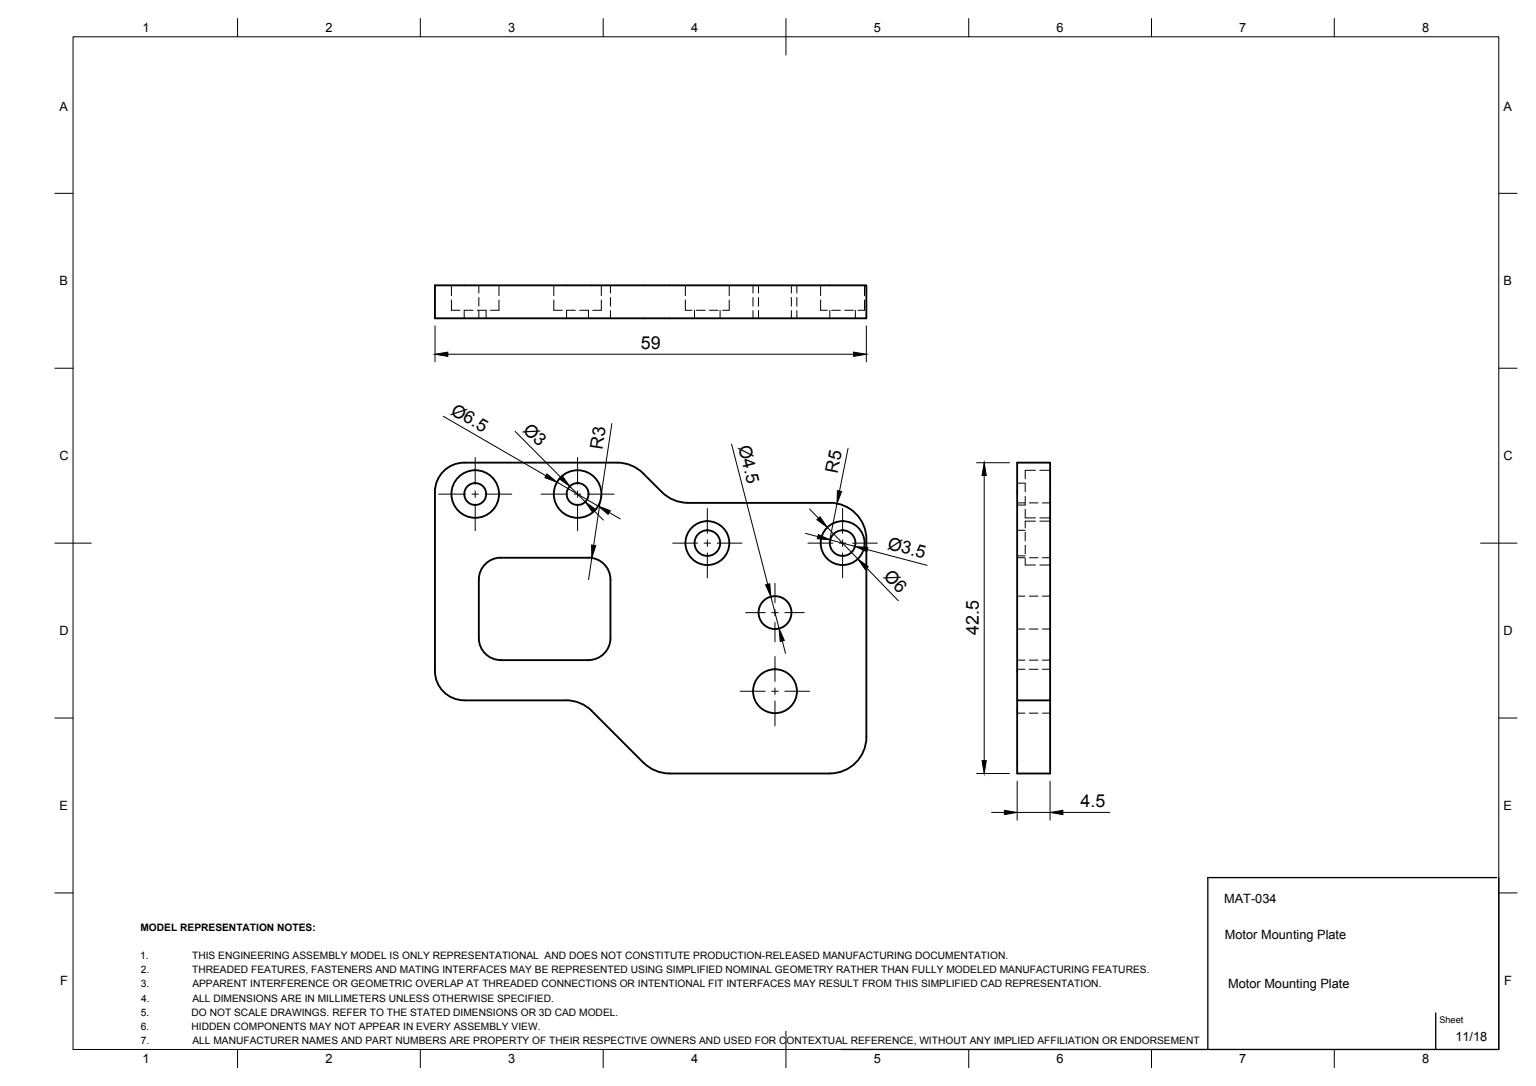
ISO-10303-21;
HEADER;
/* Generated by software containing ST-Developer
 * from STEP Tools, Inc. (www.steptools.com) 
 */

FILE_DESCRIPTION(
/* description */ ('STEP AP214'),
/* implementation_level */ '2;1');

FILE_NAME(
/* name */ 'Motor Mounting Plate.step',
/* time_stamp */ '2026-11-14T09:24:36-08:00',
/* author */ (''),
/* organization */ (''),
/* preprocessor_version */ 'ST-DEVELOPER v20.2',
/* originating_system */ 'Autodesk Translation Framework v15.17.0.0',
/* authorisation */ '');

FILE_SCHEMA (('AUTOMOTIVE_DESIGN { 1 0 10303 214 3 1 1 }'));
ENDSEC;

DATA;
#10=MECHANICAL_DESIGN_GEOMETRIC_PRESENTATION_REPRESENTATION('',(#207),#18867);
#175=SHAPE_REPRESENTATION_RELATIONSHIP('SRR','None',#18939,#191);
#191=ADVANCED_BREP_SHAPE_REPRESENTATION('',(#231),#18855);
#207=STYLED_ITEM('',(#19026),#231);
#231=MANIFOLD_SOLID_BREP('Body1',#10962);
#301=FACE_BOUND('',#1568,.T.);
#302=FACE_BOUND('',#1569,.T.);
#303=FACE_BOUND('',#1570,.T.);
#304=FACE_BOUND('',#1571,.T.);
#305=FACE_BOUND('',#1572,.T.);
#306=FACE_BOUND('',#1573,.T.);
#307=FACE_BOUND('',#1574,.T.);
#308=FACE_BOUND('',#1576,.T.);
#309=FACE_BOUND('',#1578,.T.);
#310=FACE_BOUND('',#1580,.T.);
#311=FACE_BOUND('',#1581,.T.);
#312=FACE_BOUND('',#1582,.T.);
#313=FACE_BOUND('',#1583,.T.);
#314=FACE_BOUND('',#1584,.T.);
#315=FACE_BOUND('',#1585,.T.);
#316=FACE_BOUND('',#1586,.T.);
#317=FACE_BOUND('',#1588,.T.);
#318=FACE_BOUND('',#1590,.T.);
#495=PLANE('',#11457);
#496=PLANE('',#11458);
#497=PLANE('',#11459);
#498=PLANE('',#11466);
#499=PLANE('',#11470);
#500=PLANE('',#11474);
#501=PLANE('',#11478);
#502=PLANE('',#11482);
#503=PLANE('',#11483);
#504=PLANE('',#11484);
#505=PLANE('',#11485);
#506=PLANE('',#11486);
#507=PLANE('',#11505);
#508=PLANE('',#11506);
#509=PLANE('',#11507);
#510=PLANE('',#11508);
#511=PLANE('',#11509);
#512=PLANE('',#11510);
#887=FACE_OUTER_BOUND('',#1533,.T.);
#888=FACE_OUTER_BOUND('',#1534,.T.);
#889=FACE_OUTER_BOUND('',#1535,.T.);
#890=FACE_OUTER_BOUND('',#1536,.T.);
#891=FACE_OUTER_BOUND('',#1537,.T.);
#892=FACE_OUTER_BOUND('',#1538,.T.);
#893=FACE_OUTER_BOUND('',#1539,.T.);
#894=FACE_OUTER_BOUND('',#1540,.T.);
#895=FACE_OUTER_BOUND('',#1541,.T.);
#896=FACE_OUTER_BOUND('',#1542,.T.);
#897=FACE_OUTER_BOUND('',#1543,.T.);
#898=FACE_OUTER_BOUND('',#1544,.T.);
#899=FACE_OUTER_BOUND('',#1545,.T.);
#900=FACE_OUTER_BOUND('',#1546,.T.);
#901=FACE_OUTER_BOUND('',#1547,.T.);
#902=FACE_OUTER_BOUND('',#1548,.T.);
#903=FACE_OUTER_BOUND('',#1549,.T.);
#904=FACE_OUTER_BOUND('',#1550,.T.);
#905=FACE_OUTER_BOUND('',#1551,.T.);
#906=FACE_OUTER_BOUND('',#1552,.T.);
#907=FACE_OUTER_BOUND('',#1553,.T.);
#908=FACE_OUTER_BOUND('',#1554,.T.);
#909=FACE_OUTER_BOUND('',#1555,.T.);
#910=FACE_OUTER_BOUND('',#1556,.T.);
#911=FACE_OUTER_BOUND('',#1557,.T.);
#912=FACE_OUTER_BOUND('',#1558,.T.);
#913=FACE_OUTER_BOUND('',#1559,.T.);
#914=FACE_OUTER_BOUND('',#1560,.T.);
#915=FACE_OUTER_BOUND('',#1561,.T.);
#916=FACE_OUTER_BOUND('',#1562,.T.);
#917=FACE_OUTER_BOUND('',#1563,.T.);
#918=FACE_OUTER_BOUND('',#1564,.T.);
#919=FACE_OUTER_BOUND('',#1565,.T.);
#920=FACE_OUTER_BOUND('',#1566,.T.);
#921=FACE_OUTER_BOUND('',#1567,.T.);
#922=FACE_OUTER_BOUND('',#1575,.T.);
#923=FACE_OUTER_BOUND('',#1577,.T.);
#924=FACE_OUTER_BOUND('',#1579,.T.);
#925=FACE_OUTER_BOUND('',#1587,.T.);
#926=FACE_OUTER_BOUND('',#1589,.T.);
#1533=EDGE_LOOP('',(#7916,#7917,#7918,#7919));
#1534=EDGE_LOOP('',(#7920,#7921,#7922,#7923));
#1535=EDGE_LOOP('',(#7924,#7925,#7926,#7927));
#1536=EDGE_LOOP('',(#7928,#7929,#7930,#7931));
#1537=EDGE_LOOP('',(#7932,#7933,#7934,#7935));
#1538=EDGE_LOOP('',(#7936,#7937,#7938,#7939));
#1539=EDGE_LOOP('',(#7940,#7941,#7942,#7943));
#1540=EDGE_LOOP('',(#7944,#7945,#7946,#7947));
#1541=EDGE_LOOP('',(#7948,#7949,#7950,#7951));
#1542=EDGE_LOOP('',(#7952,#7953,#7954,#7955));
#1543=EDGE_LOOP('',(#7956,#7957,#7958,#7959));
#1544=EDGE_LOOP('',(#7960,#7961,#7962,#7963));
#1545=EDGE_LOOP('',(#7964,#7965,#7966,#7967));
#1546=EDGE_LOOP('',(#7968,#7969,#7970,#7971));
#1547=EDGE_LOOP('',(#7972,#7973,#7974,#7975));
#1548=EDGE_LOOP('',(#7976,#7977,#7978,#7979));
#1549=EDGE_LOOP('',(#7980,#7981,#7982,#7983));
#1550=EDGE_LOOP('',(#7984,#7985,#7986,#7987));
#1551=EDGE_LOOP('',(#7988,#7989,#7990,#7991));
#1552=EDGE_LOOP('',(#7992,#7993,#7994,#7995));
#1553=EDGE_LOOP('',(#7996,#7997,#7998,#7999));
#1554=EDGE_LOOP('',(#8000,#8001,#8002,#8003));
#1555=EDGE_LOOP('',(#8004,#8005,#8006,#8007));
#1556=EDGE_LOOP('',(#8008,#8009,#8010,#8011));
#1557=EDGE_LOOP('',(#8012,#8013,#8014,#8015));
#1558=EDGE_LOOP('',(#8016,#8017,#8018,#8019));
#1559=EDGE_LOOP('',(#8020,#8021,#8022,#8023));
#1560=EDGE_LOOP('',(#8024,#8025,#8026,#8027));
#1561=EDGE_LOOP('',(#8028,#8029,#8030,#8031));
#1562=EDGE_LOOP('',(#8032,#8033,#8034,#8035));
#1563=EDGE_LOOP('',(#8036,#8037,#8038,#8039));
#1564=EDGE_LOOP('',(#8040,#8041,#8042,#8043));
#1565=EDGE_LOOP('',(#8044,#8045,#8046,#8047));
#1566=EDGE_LOOP('',(#8048,#8049,#8050,#8051));
#1567=EDGE_LOOP('',(#8052,#8053,#8054,#8055,#8056,#8057,#8058,#8059,#8060,
#8061,#8062,#8063,#8064,#8065,#8066,#8067));
#1568=EDGE_LOOP('',(#8068,#8069,#8070,#8071,#8072,#8073,#8074,#8075));
#1569=EDGE_LOOP('',(#8076));
#1570=EDGE_LOOP('',(#8077));
#1571=EDGE_LOOP('',(#8078));
#1572=EDGE_LOOP('',(#8079));
#1573=EDGE_LOOP('',(#8080));
#1574=EDGE_LOOP('',(#8081));
#1575=EDGE_LOOP('',(#8082));
#1576=EDGE_LOOP('',(#8083));
#1577=EDGE_LOOP('',(#8084));
#1578=EDGE_LOOP('',(#8085));
#1579=EDGE_LOOP('',(#8086,#8087,#8088,#8089,#8090,#8091,#8092,#8093,#8094,
#8095,#8096,#8097,#8098,#8099,#8100,#8101));
#1580=EDGE_LOOP('',(#8102));
#1581=EDGE_LOOP('',(#8103));
#1582=EDGE_LOOP('',(#8104));
#1583=EDGE_LOOP('',(#8105));
#1584=EDGE_LOOP('',(#8106));
#1585=EDGE_LOOP('',(#8107));
#1586=EDGE_LOOP('',(#8108,#8109,#8110,#8111,#8112,#8113,#8114,#8115));
#1587=EDGE_LOOP('',(#8116));
#1588=EDGE_LOOP('',(#8117));
#1589=EDGE_LOOP('',(#8118));
#1590=EDGE_LOOP('',(#8119));
#2351=LINE('',#16449,#3365);
#2352=LINE('',#16455,#3366);
#2353=LINE('',#16461,#3367);
#2354=LINE('',#16467,#3368);
#2355=LINE('',#16473,#3369);
#2356=LINE('',#16479,#3370);
#2357=LINE('',#16485,#3371);
#2358=LINE('',#16491,#3372);
#2359=LINE('',#16497,#3373);
#2360=LINE('',#16503,#3374);
#2361=LINE('',#16508,#3375);
#2362=LINE('',#16510,#3376);
#2363=LINE('',#16512,#3377);
#2364=LINE('',#16513,#3378);
#2365=LINE('',#16517,#3379);
#2366=LINE('',#16519,#3380);
#2367=LINE('',#16521,#3381);
#2368=LINE('',#16522,#3382);
#2369=LINE('',#16526,#3383);
#2370=LINE('',#16528,#3384);
#2371=LINE('',#16530,#3385);
#2372=LINE('',#16531,#3386);
#2373=LINE('',#16541,#3387);
#2374=LINE('',#16543,#3388);
#2375=LINE('',#16545,#3389);
#2376=LINE('',#16546,#3390);
#2377=LINE('',#16551,#3391);
#2378=LINE('',#16555,#3392);
#2379=LINE('',#16557,#3393);
#2380=LINE('',#16558,#3394);
#2381=LINE('',#16563,#3395);
#2382=LINE('',#16567,#3396);
#2383=LINE('',#16569,#3397);
#2384=LINE('',#16570,#3398);
#2385=LINE('',#16575,#3399);
#2386=LINE('',#16579,#3400);
#2387=LINE('',#16581,#3401);
#2388=LINE('',#16582,#3402);
#2389=LINE('',#16589,#3403);
#2390=LINE('',#16591,#3404);
#2391=LINE('',#16593,#3405);
#2392=LINE('',#16594,#3406);
#2393=LINE('',#16598,#3407);
#2394=LINE('',#16600,#3408);
#2395=LINE('',#16602,#3409);
#2396=LINE('',#16603,#3410);
#2397=LINE('',#16607,#3411);
#2398=LINE('',#16609,#3412);
#2399=LINE('',#16611,#3413);
#2400=LINE('',#16612,#3414);
#2401=LINE('',#16616,#3415);
#2402=LINE('',#16618,#3416);
#2403=LINE('',#16620,#3417);
#2404=LINE('',#16621,#3418);
#2405=LINE('',#16625,#3419);
#2406=LINE('',#16627,#3420);
#2407=LINE('',#16629,#3421);
#2408=LINE('',#16630,#3422);
#3365=VECTOR('',#13147,3.);
#3366=VECTOR('',#13154,3.);
#3367=VECTOR('',#13161,3.25);
#3368=VECTOR('',#13168,3.25);
#3369=VECTOR('',#13175,2.25);
#3370=VECTOR('',#13182,1.75);
#3371=VECTOR('',#13189,1.75);
#3372=VECTOR('',#13196,3.);
#3373=VECTOR('',#13203,1.5);
#3374=VECTOR('',#13210,1.5);
#3375=VECTOR('',#13215,1000.);
#3376=VECTOR('',#13216,1000.);
#3377=VECTOR('',#13217,1000.);
#3378=VECTOR('',#13218,1000.);
#3379=VECTOR('',#13221,1000.);
#3380=VECTOR('',#13222,1000.);
#3381=VECTOR('',#13223,1000.);
#3382=VECTOR('',#13224,1000.);
#3383=VECTOR('',#13227,1000.);
#3384=VECTOR('',#13228,1000.);
#3385=VECTOR('',#13229,1000.);
#3386=VECTOR('',#13230,1000.);
#3387=VECTOR('',#13245,1000.);
#3388=VECTOR('',#13246,1000.);
#3389=VECTOR('',#13247,1000.);
#3390=VECTOR('',#13248,1000.);
#3391=VECTOR('',#13253,1000.);
#3392=VECTOR('',#13258,1000.);
#3393=VECTOR('',#13259,1000.);
#3394=VECTOR('',#13260,1000.);
#3395=VECTOR('',#13265,1000.);
#3396=VECTOR('',#13270,1000.);
#3397=VECTOR('',#13271,1000.);
#3398=VECTOR('',#13272,1000.);
#3399=VECTOR('',#13277,1000.);
#3400=VECTOR('',#13282,1000.);
#3401=VECTOR('',#13283,1000.);
#3402=VECTOR('',#13284,1000.);
#3403=VECTOR('',#13293,1000.);
#3404=VECTOR('',#13294,1000.);
#3405=VECTOR('',#13295,1000.);
#3406=VECTOR('',#13296,1000.);
#3407=VECTOR('',#13299,1000.);
#3408=VECTOR('',#13300,1000.);
#3409=VECTOR('',#13301,1000.);
#3410=VECTOR('',#13302,1000.);
#3411=VECTOR('',#13305,1000.);
#3412=VECTOR('',#13306,1000.);
#3413=VECTOR('',#13307,1000.);
#3414=VECTOR('',#13308,1000.);
#3415=VECTOR('',#13311,1000.);
#3416=VECTOR('',#13312,1000.);
#3417=VECTOR('',#13313,1000.);
#3418=VECTOR('',#13314,1000.);
#3419=VECTOR('',#13317,1000.);
#3420=VECTOR('',#13318,1000.);
#3421=VECTOR('',#13319,1000.);
#3422=VECTOR('',#13320,1000.);
#4171=CIRCLE('',#11428,3.);
#4172=CIRCLE('',#11429,3.);
#4173=CIRCLE('',#11431,3.);
#4174=CIRCLE('',#11432,3.);
#4175=CIRCLE('',#11434,3.25);
#4176=CIRCLE('',#11435,3.25);
#4177=CIRCLE('',#11437,3.25);
#4178=CIRCLE('',#11438,3.25);
#4179=CIRCLE('',#11440,2.25);
#4180=CIRCLE('',#11441,2.25);
#4181=CIRCLE('',#11443,1.75);
#4182=CIRCLE('',#11444,1.75);
#4183=CIRCLE('',#11446,1.75);
#4184=CIRCLE('',#11447,1.75);
#4185=CIRCLE('',#11449,3.);
#4186=CIRCLE('',#11450,3.);
#4187=CIRCLE('',#11452,1.5);
#4188=CIRCLE('',#11453,1.5);
#4189=CIRCLE('',#11455,1.5);
#4190=CIRCLE('',#11456,1.5);
#4191=CIRCLE('',#11461,4.);
#4192=CIRCLE('',#11462,4.);
#4193=CIRCLE('',#11464,4.);
#4194=CIRCLE('',#11465,4.);
#4195=CIRCLE('',#11468,3.);
#4196=CIRCLE('',#11469,3.);
#4197=CIRCLE('',#11472,3.);
#4198=CIRCLE('',#11473,3.);
#4199=CIRCLE('',#11476,3.);
#4200=CIRCLE('',#11477,3.);
#4201=CIRCLE('',#11480,3.);
#4202=CIRCLE('',#11481,3.);
#4203=CIRCLE('',#11488,5.);
#4204=CIRCLE('',#11489,5.);
#4205=CIRCLE('',#11491,5.);
#4206=CIRCLE('',#11492,5.);
#4207=CIRCLE('',#11494,5.);
#4208=CIRCLE('',#11495,5.);
#4209=CIRCLE('',#11497,5.);
#4210=CIRCLE('',#11498,5.);
#4211=CIRCLE('',#11500,5.);
#4212=CIRCLE('',#11501,5.);
#4213=CIRCLE('',#11503,5.);
#4214=CIRCLE('',#11504,5.);
#4842=VERTEX_POINT('',#16446);
#4843=VERTEX_POINT('',#16448);
#4844=VERTEX_POINT('',#16452);
#4845=VERTEX_POINT('',#16454);
#4846=VERTEX_POINT('',#16458);
#4847=VERTEX_POINT('',#16460);
#4848=VERTEX_POINT('',#16464);
#4849=VERTEX_POINT('',#16466);
#4850=VERTEX_POINT('',#16470);
#4851=VERTEX_POINT('',#16472);
#4852=VERTEX_POINT('',#16476);
#4853=VERTEX_POINT('',#16478);
#4854=VERTEX_POINT('',#16482);
#4855=VERTEX_POINT('',#16484);
#4856=VERTEX_POINT('',#16488);
#4857=VERTEX_POINT('',#16490);
#4858=VERTEX_POINT('',#16494);
#4859=VERTEX_POINT('',#16496);
#4860=VERTEX_POINT('',#16500);
#4861=VERTEX_POINT('',#16502);
#4862=VERTEX_POINT('',#16506);
#4863=VERTEX_POINT('',#16507);
#4864=VERTEX_POINT('',#16509);
#4865=VERTEX_POINT('',#16511);
#4866=VERTEX_POINT('',#16515);
#4867=VERTEX_POINT('',#16516);
#4868=VERTEX_POINT('',#16518);
#4869=VERTEX_POINT('',#16520);
#4870=VERTEX_POINT('',#16524);
#4871=VERTEX_POINT('',#16525);
#4872=VERTEX_POINT('',#16527);
#4873=VERTEX_POINT('',#16529);
#4874=VERTEX_POINT('',#16539);
#4875=VERTEX_POINT('',#16540);
#4876=VERTEX_POINT('',#16542);
#4877=VERTEX_POINT('',#16544);
#4878=VERTEX_POINT('',#16548);
#4879=VERTEX_POINT('',#16550);
#4880=VERTEX_POINT('',#16554);
#4881=VERTEX_POINT('',#16556);
#4882=VERTEX_POINT('',#16560);
#4883=VERTEX_POINT('',#16562);
#4884=VERTEX_POINT('',#16566);
#4885=VERTEX_POINT('',#16568);
#4886=VERTEX_POINT('',#16572);
#4887=VERTEX_POINT('',#16574);
#4888=VERTEX_POINT('',#16578);
#4889=VERTEX_POINT('',#16580);
#4890=VERTEX_POINT('',#16587);
#4891=VERTEX_POINT('',#16588);
#4892=VERTEX_POINT('',#16590);
#4893=VERTEX_POINT('',#16592);
#4894=VERTEX_POINT('',#16596);
#4895=VERTEX_POINT('',#16597);
#4896=VERTEX_POINT('',#16599);
#4897=VERTEX_POINT('',#16601);
#4898=VERTEX_POINT('',#16605);
#4899=VERTEX_POINT('',#16606);
#4900=VERTEX_POINT('',#16608);
#4901=VERTEX_POINT('',#16610);
#4902=VERTEX_POINT('',#16614);
#4903=VERTEX_POINT('',#16615);
#4904=VERTEX_POINT('',#16617);
#4905=VERTEX_POINT('',#16619);
#4906=VERTEX_POINT('',#16623);
#4907=VERTEX_POINT('',#16624);
#4908=VERTEX_POINT('',#16626);
#4909=VERTEX_POINT('',#16628);
#5991=EDGE_CURVE('',#4842,#4842,#4171,.T.);
#5992=EDGE_CURVE('',#4842,#4843,#2351,.T.);
#5993=EDGE_CURVE('',#4843,#4843,#4172,.T.);
#5994=EDGE_CURVE('',#4844,#4844,#4173,.T.);
#5995=EDGE_CURVE('',#4844,#4845,#2352,.T.);
#5996=EDGE_CURVE('',#4845,#4845,#4174,.T.);
#5997=EDGE_CURVE('',#4846,#4846,#4175,.T.);
#5998=EDGE_CURVE('',#4846,#4847,#2353,.T.);
#5999=EDGE_CURVE('',#4847,#4847,#4176,.T.);
#6000=EDGE_CURVE('',#4848,#4848,#4177,.T.);
#6001=EDGE_CURVE('',#4848,#4849,#2354,.T.);
#6002=EDGE_CURVE('',#4849,#4849,#4178,.T.);
#6003=EDGE_CURVE('',#4850,#4850,#4179,.T.);
#6004=EDGE_CURVE('',#4850,#4851,#2355,.T.);
#6005=EDGE_CURVE('',#4851,#4851,#4180,.T.);
#6006=EDGE_CURVE('',#4852,#4852,#4181,.T.);
#6007=EDGE_CURVE('',#4852,#4853,#2356,.T.);
#6008=EDGE_CURVE('',#4853,#4853,#4182,.T.);
#6009=EDGE_CURVE('',#4854,#4854,#4183,.T.);
#6010=EDGE_CURVE('',#4854,#4855,#2357,.T.);
#6011=EDGE_CURVE('',#4855,#4855,#4184,.T.);
#6012=EDGE_CURVE('',#4856,#4856,#4185,.T.);
#6013=EDGE_CURVE('',#4856,#4857,#2358,.T.);
#6014=EDGE_CURVE('',#4857,#4857,#4186,.T.);
#6015=EDGE_CURVE('',#4858,#4858,#4187,.T.);
#6016=EDGE_CURVE('',#4858,#4859,#2359,.T.);
#6017=EDGE_CURVE('',#4859,#4859,#4188,.T.);
#6018=EDGE_CURVE('',#4860,#4860,#4189,.T.);
#6019=EDGE_CURVE('',#4860,#4861,#2360,.T.);
#6020=EDGE_CURVE('',#4861,#4861,#4190,.T.);
#6021=EDGE_CURVE('',#4862,#4863,#2361,.T.);
#6022=EDGE_CURVE('',#4862,#4864,#2362,.T.);
#6023=EDGE_CURVE('',#4865,#4864,#2363,.T.);
#6024=EDGE_CURVE('',#4865,#4863,#2364,.T.);
#6025=EDGE_CURVE('',#4866,#4867,#2365,.T.);
#6026=EDGE_CURVE('',#4866,#4868,#2366,.T.);
#6027=EDGE_CURVE('',#4869,#4868,#2367,.T.);
#6028=EDGE_CURVE('',#4869,#4867,#2368,.T.);
#6029=EDGE_CURVE('',#4870,#4871,#2369,.T.);
#6030=EDGE_CURVE('',#4870,#4872,#2370,.T.);
#6031=EDGE_CURVE('',#4873,#4872,#2371,.T.);
#6032=EDGE_CURVE('',#4873,#4871,#2372,.T.);
#6033=EDGE_CURVE('',#4871,#4866,#4191,.T.);
#6034=EDGE_CURVE('',#4868,#4873,#4192,.T.);
#6035=EDGE_CURVE('',#4867,#4862,#4193,.T.);
#6036=EDGE_CURVE('',#4864,#4869,#4194,.T.);
#6037=EDGE_CURVE('',#4874,#4875,#2373,.T.);
#6038=EDGE_CURVE('',#4874,#4876,#2374,.T.);
#6039=EDGE_CURVE('',#4876,#4877,#2375,.T.);
#6040=EDGE_CURVE('',#4875,#4877,#2376,.T.);
#6041=EDGE_CURVE('',#4878,#4876,#4195,.T.);
#6042=EDGE_CURVE('',#4878,#4879,#2377,.T.);
#6043=EDGE_CURVE('',#4879,#4877,#4196,.T.);
#6044=EDGE_CURVE('',#4878,#4880,#2378,.T.);
#6045=EDGE_CURVE('',#4880,#4881,#2379,.T.);
#6046=EDGE_CURVE('',#4879,#4881,#2380,.T.);
#6047=EDGE_CURVE('',#4882,#4880,#4197,.T.);
#6048=EDGE_CURVE('',#4882,#4883,#2381,.T.);
#6049=EDGE_CURVE('',#4883,#4881,#4198,.T.);
#6050=EDGE_CURVE('',#4884,#4882,#2382,.T.);
#6051=EDGE_CURVE('',#4884,#4885,#2383,.T.);
#6052=EDGE_CURVE('',#4885,#4883,#2384,.T.);
#6053=EDGE_CURVE('',#4886,#4884,#4199,.T.);
#6054=EDGE_CURVE('',#4886,#4887,#2385,.T.);
#6055=EDGE_CURVE('',#4887,#4885,#4200,.T.);
#6056=EDGE_CURVE('',#4888,#4886,#2386,.T.);
#6057=EDGE_CURVE('',#4888,#4889,#2387,.T.);
#6058=EDGE_CURVE('',#4889,#4887,#2388,.T.);
#6059=EDGE_CURVE('',#4874,#4888,#4201,.T.);
#6060=EDGE_CURVE('',#4875,#4889,#4202,.T.);
#6061=EDGE_CURVE('',#4890,#4891,#2389,.T.);
#6062=EDGE_CURVE('',#4892,#4891,#2390,.T.);
#6063=EDGE_CURVE('',#4892,#4893,#2391,.T.);
#6064=EDGE_CURVE('',#4890,#4893,#2392,.T.);
#6065=EDGE_CURVE('',#4894,#4895,#2393,.T.);
#6066=EDGE_CURVE('',#4896,#4895,#2394,.T.);
#6067=EDGE_CURVE('',#4896,#4897,#2395,.T.);
#6068=EDGE_CURVE('',#4894,#4897,#2396,.T.);
#6069=EDGE_CURVE('',#4898,#4899,#2397,.T.);
#6070=EDGE_CURVE('',#4900,#4899,#2398,.T.);
#6071=EDGE_CURVE('',#4900,#4901,#2399,.T.);
#6072=EDGE_CURVE('',#4898,#4901,#2400,.T.);
#6073=EDGE_CURVE('',#4902,#4903,#2401,.T.);
#6074=EDGE_CURVE('',#4904,#4903,#2402,.T.);
#6075=EDGE_CURVE('',#4904,#4905,#2403,.T.);
#6076=EDGE_CURVE('',#4902,#4905,#2404,.T.);
#6077=EDGE_CURVE('',#4906,#4907,#2405,.T.);
#6078=EDGE_CURVE('',#4908,#4907,#2406,.T.);
#6079=EDGE_CURVE('',#4908,#4909,#2407,.T.);
#6080=EDGE_CURVE('',#4906,#4909,#2408,.T.);
#6081=EDGE_CURVE('',#4863,#4908,#4203,.T.);
#6082=EDGE_CURVE('',#4909,#4865,#4204,.T.);
#6083=EDGE_CURVE('',#4907,#4904,#4205,.T.);
#6084=EDGE_CURVE('',#4905,#4906,#4206,.T.);
#6085=EDGE_CURVE('',#4903,#4900,#4207,.T.);
#6086=EDGE_CURVE('',#4901,#4902,#4208,.T.);
#6087=EDGE_CURVE('',#4899,#4892,#4209,.T.);
#6088=EDGE_CURVE('',#4893,#4898,#4210,.T.);
#6089=EDGE_CURVE('',#4891,#4896,#4211,.T.);
#6090=EDGE_CURVE('',#4897,#4890,#4212,.T.);
#6091=EDGE_CURVE('',#4895,#4870,#4213,.T.);
#6092=EDGE_CURVE('',#4872,#4894,#4214,.T.);
#7916=ORIENTED_EDGE('',*,*,#5991,.F.);
#7917=ORIENTED_EDGE('',*,*,#5992,.T.);
#7918=ORIENTED_EDGE('',*,*,#5993,.T.);
#7919=ORIENTED_EDGE('',*,*,#5992,.F.);
#7920=ORIENTED_EDGE('',*,*,#5994,.F.);
#7921=ORIENTED_EDGE('',*,*,#5995,.T.);
#7922=ORIENTED_EDGE('',*,*,#5996,.T.);
#7923=ORIENTED_EDGE('',*,*,#5995,.F.);
#7924=ORIENTED_EDGE('',*,*,#5997,.F.);
#7925=ORIENTED_EDGE('',*,*,#5998,.T.);
#7926=ORIENTED_EDGE('',*,*,#5999,.T.);
#7927=ORIENTED_EDGE('',*,*,#5998,.F.);
#7928=ORIENTED_EDGE('',*,*,#6000,.F.);
#7929=ORIENTED_EDGE('',*,*,#6001,.T.);
#7930=ORIENTED_EDGE('',*,*,#6002,.T.);
#7931=ORIENTED_EDGE('',*,*,#6001,.F.);
#7932=ORIENTED_EDGE('',*,*,#6003,.F.);
#7933=ORIENTED_EDGE('',*,*,#6004,.T.);
#7934=ORIENTED_EDGE('',*,*,#6005,.F.);
#7935=ORIENTED_EDGE('',*,*,#6004,.F.);
#7936=ORIENTED_EDGE('',*,*,#6006,.F.);
#7937=ORIENTED_EDGE('',*,*,#6007,.T.);
#7938=ORIENTED_EDGE('',*,*,#6008,.T.);
#7939=ORIENTED_EDGE('',*,*,#6007,.F.);
#7940=ORIENTED_EDGE('',*,*,#6009,.F.);
#7941=ORIENTED_EDGE('',*,*,#6010,.T.);
#7942=ORIENTED_EDGE('',*,*,#6011,.T.);
#7943=ORIENTED_EDGE('',*,*,#6010,.F.);
#7944=ORIENTED_EDGE('',*,*,#6012,.F.);
#7945=ORIENTED_EDGE('',*,*,#6013,.T.);
#7946=ORIENTED_EDGE('',*,*,#6014,.T.);
#7947=ORIENTED_EDGE('',*,*,#6013,.F.);
#7948=ORIENTED_EDGE('',*,*,#6015,.F.);
#7949=ORIENTED_EDGE('',*,*,#6016,.T.);
#7950=ORIENTED_EDGE('',*,*,#6017,.T.);
#7951=ORIENTED_EDGE('',*,*,#6016,.F.);
#7952=ORIENTED_EDGE('',*,*,#6018,.F.);
#7953=ORIENTED_EDGE('',*,*,#6019,.T.);
#7954=ORIENTED_EDGE('',*,*,#6020,.T.);
#7955=ORIENTED_EDGE('',*,*,#6019,.F.);
#7956=ORIENTED_EDGE('',*,*,#6021,.F.);
#7957=ORIENTED_EDGE('',*,*,#6022,.T.);
#7958=ORIENTED_EDGE('',*,*,#6023,.F.);
#7959=ORIENTED_EDGE('',*,*,#6024,.T.);
#7960=ORIENTED_EDGE('',*,*,#6025,.F.);
#7961=ORIENTED_EDGE('',*,*,#6026,.T.);
#7962=ORIENTED_EDGE('',*,*,#6027,.F.);
#7963=ORIENTED_EDGE('',*,*,#6028,.T.);
#7964=ORIENTED_EDGE('',*,*,#6029,.F.);
#7965=ORIENTED_EDGE('',*,*,#6030,.T.);
#7966=ORIENTED_EDGE('',*,*,#6031,.F.);
#7967=ORIENTED_EDGE('',*,*,#6032,.T.);
#7968=ORIENTED_EDGE('',*,*,#6026,.F.);
#7969=ORIENTED_EDGE('',*,*,#6033,.F.);
#7970=ORIENTED_EDGE('',*,*,#6032,.F.);
#7971=ORIENTED_EDGE('',*,*,#6034,.F.);
#7972=ORIENTED_EDGE('',*,*,#6022,.F.);
#7973=ORIENTED_EDGE('',*,*,#6035,.F.);
#7974=ORIENTED_EDGE('',*,*,#6028,.F.);
#7975=ORIENTED_EDGE('',*,*,#6036,.F.);
#7976=ORIENTED_EDGE('',*,*,#6037,.F.);
#7977=ORIENTED_EDGE('',*,*,#6038,.T.);
#7978=ORIENTED_EDGE('',*,*,#6039,.T.);
#7979=ORIENTED_EDGE('',*,*,#6040,.F.);
#7980=ORIENTED_EDGE('',*,*,#6041,.F.);
#7981=ORIENTED_EDGE('',*,*,#6042,.T.);
#7982=ORIENTED_EDGE('',*,*,#6043,.T.);
#7983=ORIENTED_EDGE('',*,*,#6039,.F.);
#7984=ORIENTED_EDGE('',*,*,#6042,.F.);
#7985=ORIENTED_EDGE('',*,*,#6044,.T.);
#7986=ORIENTED_EDGE('',*,*,#6045,.T.);
#7987=ORIENTED_EDGE('',*,*,#6046,.F.);
#7988=ORIENTED_EDGE('',*,*,#6047,.F.);
#7989=ORIENTED_EDGE('',*,*,#6048,.T.);
#7990=ORIENTED_EDGE('',*,*,#6049,.T.);
#7991=ORIENTED_EDGE('',*,*,#6045,.F.);
#7992=ORIENTED_EDGE('',*,*,#6050,.F.);
#7993=ORIENTED_EDGE('',*,*,#6051,.T.);
#7994=ORIENTED_EDGE('',*,*,#6052,.T.);
#7995=ORIENTED_EDGE('',*,*,#6048,.F.);
#7996=ORIENTED_EDGE('',*,*,#6053,.F.);
#7997=ORIENTED_EDGE('',*,*,#6054,.T.);
#7998=ORIENTED_EDGE('',*,*,#6055,.T.);
#7999=ORIENTED_EDGE('',*,*,#6051,.F.);
#8000=ORIENTED_EDGE('',*,*,#6056,.F.);
#8001=ORIENTED_EDGE('',*,*,#6057,.T.);
#8002=ORIENTED_EDGE('',*,*,#6058,.T.);
#8003=ORIENTED_EDGE('',*,*,#6054,.F.);
#8004=ORIENTED_EDGE('',*,*,#6059,.F.);
#8005=ORIENTED_EDGE('',*,*,#6037,.T.);
#8006=ORIENTED_EDGE('',*,*,#6060,.T.);
#8007=ORIENTED_EDGE('',*,*,#6057,.F.);
#8008=ORIENTED_EDGE('',*,*,#6061,.T.);
#8009=ORIENTED_EDGE('',*,*,#6062,.F.);
#8010=ORIENTED_EDGE('',*,*,#6063,.T.);
#8011=ORIENTED_EDGE('',*,*,#6064,.F.);
#8012=ORIENTED_EDGE('',*,*,#6065,.T.);
#8013=ORIENTED_EDGE('',*,*,#6066,.F.);
#8014=ORIENTED_EDGE('',*,*,#6067,.T.);
#8015=ORIENTED_EDGE('',*,*,#6068,.F.);
#8016=ORIENTED_EDGE('',*,*,#6069,.T.);
#8017=ORIENTED_EDGE('',*,*,#6070,.F.);
#8018=ORIENTED_EDGE('',*,*,#6071,.T.);
#8019=ORIENTED_EDGE('',*,*,#6072,.F.);
#8020=ORIENTED_EDGE('',*,*,#6073,.T.);
#8021=ORIENTED_EDGE('',*,*,#6074,.F.);
#8022=ORIENTED_EDGE('',*,*,#6075,.T.);
#8023=ORIENTED_EDGE('',*,*,#6076,.F.);
#8024=ORIENTED_EDGE('',*,*,#6077,.T.);
#8025=ORIENTED_EDGE('',*,*,#6078,.F.);
#8026=ORIENTED_EDGE('',*,*,#6079,.T.);
#8027=ORIENTED_EDGE('',*,*,#6080,.F.);
#8028=ORIENTED_EDGE('',*,*,#6079,.F.);
#8029=ORIENTED_EDGE('',*,*,#6081,.F.);
#8030=ORIENTED_EDGE('',*,*,#6024,.F.);
#8031=ORIENTED_EDGE('',*,*,#6082,.F.);
#8032=ORIENTED_EDGE('',*,*,#6083,.F.);
#8033=ORIENTED_EDGE('',*,*,#6077,.F.);
#8034=ORIENTED_EDGE('',*,*,#6084,.F.);
#8035=ORIENTED_EDGE('',*,*,#6075,.F.);
#8036=ORIENTED_EDGE('',*,*,#6071,.F.);
#8037=ORIENTED_EDGE('',*,*,#6085,.F.);
#8038=ORIENTED_EDGE('',*,*,#6073,.F.);
#8039=ORIENTED_EDGE('',*,*,#6086,.F.);
#8040=ORIENTED_EDGE('',*,*,#6063,.F.);
#8041=ORIENTED_EDGE('',*,*,#6087,.F.);
#8042=ORIENTED_EDGE('',*,*,#6069,.F.);
#8043=ORIENTED_EDGE('',*,*,#6088,.F.);
#8044=ORIENTED_EDGE('',*,*,#6067,.F.);
#8045=ORIENTED_EDGE('',*,*,#6089,.F.);
#8046=ORIENTED_EDGE('',*,*,#6061,.F.);
#8047=ORIENTED_EDGE('',*,*,#6090,.F.);
#8048=ORIENTED_EDGE('',*,*,#6091,.F.);
#8049=ORIENTED_EDGE('',*,*,#6065,.F.);
#8050=ORIENTED_EDGE('',*,*,#6092,.F.);
#8051=ORIENTED_EDGE('',*,*,#6030,.F.);
#8052=ORIENTED_EDGE('',*,*,#6080,.T.);
#8053=ORIENTED_EDGE('',*,*,#6082,.T.);
#8054=ORIENTED_EDGE('',*,*,#6023,.T.);
#8055=ORIENTED_EDGE('',*,*,#6036,.T.);
#8056=ORIENTED_EDGE('',*,*,#6027,.T.);
#8057=ORIENTED_EDGE('',*,*,#6034,.T.);
#8058=ORIENTED_EDGE('',*,*,#6031,.T.);
#8059=ORIENTED_EDGE('',*,*,#6092,.T.);
#8060=ORIENTED_EDGE('',*,*,#6068,.T.);
#8061=ORIENTED_EDGE('',*,*,#6090,.T.);
#8062=ORIENTED_EDGE('',*,*,#6064,.T.);
#8063=ORIENTED_EDGE('',*,*,#6088,.T.);
#8064=ORIENTED_EDGE('',*,*,#6072,.T.);
#8065=ORIENTED_EDGE('',*,*,#6086,.T.);
#8066=ORIENTED_EDGE('',*,*,#6076,.T.);
#8067=ORIENTED_EDGE('',*,*,#6084,.T.);
#8068=ORIENTED_EDGE('',*,*,#6060,.F.);
#8069=ORIENTED_EDGE('',*,*,#6040,.T.);
#8070=ORIENTED_EDGE('',*,*,#6043,.F.);
#8071=ORIENTED_EDGE('',*,*,#6046,.T.);
#8072=ORIENTED_EDGE('',*,*,#6049,.F.);
#8073=ORIENTED_EDGE('',*,*,#6052,.F.);
#8074=ORIENTED_EDGE('',*,*,#6055,.F.);
#8075=ORIENTED_EDGE('',*,*,#6058,.F.);
#8076=ORIENTED_EDGE('',*,*,#5993,.F.);
#8077=ORIENTED_EDGE('',*,*,#5996,.F.);
#8078=ORIENTED_EDGE('',*,*,#6003,.T.);
#8079=ORIENTED_EDGE('',*,*,#6014,.F.);
#8080=ORIENTED_EDGE('',*,*,#5999,.F.);
#8081=ORIENTED_EDGE('',*,*,#6002,.F.);
#8082=ORIENTED_EDGE('',*,*,#6000,.T.);
#8083=ORIENTED_EDGE('',*,*,#6020,.F.);
#8084=ORIENTED_EDGE('',*,*,#5997,.T.);
#8085=ORIENTED_EDGE('',*,*,#6017,.F.);
#8086=ORIENTED_EDGE('',*,*,#6035,.T.);
#8087=ORIENTED_EDGE('',*,*,#6021,.T.);
#8088=ORIENTED_EDGE('',*,*,#6081,.T.);
#8089=ORIENTED_EDGE('',*,*,#6078,.T.);
#8090=ORIENTED_EDGE('',*,*,#6083,.T.);
#8091=ORIENTED_EDGE('',*,*,#6074,.T.);
#8092=ORIENTED_EDGE('',*,*,#6085,.T.);
#8093=ORIENTED_EDGE('',*,*,#6070,.T.);
#8094=ORIENTED_EDGE('',*,*,#6087,.T.);
#8095=ORIENTED_EDGE('',*,*,#6062,.T.);
#8096=ORIENTED_EDGE('',*,*,#6089,.T.);
#8097=ORIENTED_EDGE('',*,*,#6066,.T.);
#8098=ORIENTED_EDGE('',*,*,#6091,.T.);
#8099=ORIENTED_EDGE('',*,*,#6029,.T.);
#8100=ORIENTED_EDGE('',*,*,#6033,.T.);
#8101=ORIENTED_EDGE('',*,*,#6025,.T.);
#8102=ORIENTED_EDGE('',*,*,#6005,.T.);
#8103=ORIENTED_EDGE('',*,*,#6006,.T.);
#8104=ORIENTED_EDGE('',*,*,#6009,.T.);
#8105=ORIENTED_EDGE('',*,*,#6012,.T.);
#8106=ORIENTED_EDGE('',*,*,#6015,.T.);
#8107=ORIENTED_EDGE('',*,*,#6018,.T.);
#8108=ORIENTED_EDGE('',*,*,#6059,.T.);
#8109=ORIENTED_EDGE('',*,*,#6056,.T.);
#8110=ORIENTED_EDGE('',*,*,#6053,.T.);
#8111=ORIENTED_EDGE('',*,*,#6050,.T.);
#8112=ORIENTED_EDGE('',*,*,#6047,.T.);
#8113=ORIENTED_EDGE('',*,*,#6044,.F.);
#8114=ORIENTED_EDGE('',*,*,#6041,.T.);
#8115=ORIENTED_EDGE('',*,*,#6038,.F.);
#8116=ORIENTED_EDGE('',*,*,#5994,.T.);
#8117=ORIENTED_EDGE('',*,*,#6008,.F.);
#8118=ORIENTED_EDGE('',*,*,#5991,.T.);
#8119=ORIENTED_EDGE('',*,*,#6011,.F.);
#10198=CYLINDRICAL_SURFACE('',#11427,3.);
#10199=CYLINDRICAL_SURFACE('',#11430,3.);
#10200=CYLINDRICAL_SURFACE('',#11433,3.25);
#10201=CYLINDRICAL_SURFACE('',#11436,3.25);
#10202=CYLINDRICAL_SURFACE('',#11439,2.25);
#10203=CYLINDRICAL_SURFACE('',#11442,1.75);
#10204=CYLINDRICAL_SURFACE('',#11445,1.75);
#10205=CYLINDRICAL_SURFACE('',#11448,3.);
#10206=CYLINDRICAL_SURFACE('',#11451,1.5);
#10207=CYLINDRICAL_SURFACE('',#11454,1.5);
#10208=CYLINDRICAL_SURFACE('',#11460,4.);
#10209=CYLINDRICAL_SURFACE('',#11463,4.);
#10210=CYLINDRICAL_SURFACE('',#11467,3.);
#10211=CYLINDRICAL_SURFACE('',#11471,3.);
#10212=CYLINDRICAL_SURFACE('',#11475,3.);
#10213=CYLINDRICAL_SURFACE('',#11479,3.);
#10214=CYLINDRICAL_SURFACE('',#11487,5.);
#10215=CYLINDRICAL_SURFACE('',#11490,5.);
#10216=CYLINDRICAL_SURFACE('',#11493,5.);
#10217=CYLINDRICAL_SURFACE('',#11496,5.);
#10218=CYLINDRICAL_SURFACE('',#11499,5.);
#10219=CYLINDRICAL_SURFACE('',#11502,5.);
#10524=ADVANCED_FACE('',(#887),#10198,.F.);
#10525=ADVANCED_FACE('',(#888),#10199,.F.);
#10526=ADVANCED_FACE('',(#889),#10200,.F.);
#10527=ADVANCED_FACE('',(#890),#10201,.F.);
#10528=ADVANCED_FACE('',(#891),#10202,.F.);
#10529=ADVANCED_FACE('',(#892),#10203,.F.);
#10530=ADVANCED_FACE('',(#893),#10204,.F.);
#10531=ADVANCED_FACE('',(#894),#10205,.F.);
#10532=ADVANCED_FACE('',(#895),#10206,.F.);
#10533=ADVANCED_FACE('',(#896),#10207,.F.);
#10534=ADVANCED_FACE('',(#897),#495,.F.);
#10535=ADVANCED_FACE('',(#898),#496,.F.);
#10536=ADVANCED_FACE('',(#899),#497,.F.);
#10537=ADVANCED_FACE('',(#900),#10208,.T.);
#10538=ADVANCED_FACE('',(#901),#10209,.T.);
#10539=ADVANCED_FACE('',(#902),#498,.T.);
#10540=ADVANCED_FACE('',(#903),#10210,.F.);
#10541=ADVANCED_FACE('',(#904),#499,.T.);
#10542=ADVANCED_FACE('',(#905),#10211,.F.);
#10543=ADVANCED_FACE('',(#906),#500,.F.);
#10544=ADVANCED_FACE('',(#907),#10212,.F.);
#10545=ADVANCED_FACE('',(#908),#501,.F.);
#10546=ADVANCED_FACE('',(#909),#10213,.F.);
#10547=ADVANCED_FACE('',(#910),#502,.T.);
#10548=ADVANCED_FACE('',(#911),#503,.T.);
#10549=ADVANCED_FACE('',(#912),#504,.T.);
#10550=ADVANCED_FACE('',(#913),#505,.T.);
#10551=ADVANCED_FACE('',(#914),#506,.T.);
#10552=ADVANCED_FACE('',(#915),#10214,.T.);
#10553=ADVANCED_FACE('',(#916),#10215,.F.);
#10554=ADVANCED_FACE('',(#917),#10216,.T.);
#10555=ADVANCED_FACE('',(#918),#10217,.T.);
#10556=ADVANCED_FACE('',(#919),#10218,.T.);
#10557=ADVANCED_FACE('',(#920),#10219,.F.);
#10558=ADVANCED_FACE('',(#921,#301,#302,#303,#304,#305,#306,#307),#507,
 .T.);
#10559=ADVANCED_FACE('',(#922,#308),#508,.F.);
#10560=ADVANCED_FACE('',(#923,#309),#509,.F.);
#10561=ADVANCED_FACE('',(#924,#310,#311,#312,#313,#314,#315,#316),#510,
 .T.);
#10562=ADVANCED_FACE('',(#925,#317),#511,.F.);
#10563=ADVANCED_FACE('',(#926,#318),#512,.F.);
#10962=CLOSED_SHELL('',(#10524,#10525,#10526,#10527,#10528,#10529,#10530,
#10531,#10532,#10533,#10534,#10535,#10536,#10537,#10538,#10539,#10540,#10541,
#10542,#10543,#10544,#10545,#10546,#10547,#10548,#10549,#10550,#10551,#10552,
#10553,#10554,#10555,#10556,#10557,#10558,#10559,#10560,#10561,#10562,#10563));
#11426=AXIS2_PLACEMENT_3D('',#16444,#13141,#13142);
#11427=AXIS2_PLACEMENT_3D('',#16445,#13143,#13144);
#11428=AXIS2_PLACEMENT_3D('',#16447,#13145,#13146);
#11429=AXIS2_PLACEMENT_3D('',#16450,#13148,#13149);
#11430=AXIS2_PLACEMENT_3D('',#16451,#13150,#13151);
#11431=AXIS2_PLACEMENT_3D('',#16453,#13152,#13153);
#11432=AXIS2_PLACEMENT_3D('',#16456,#13155,#13156);
#11433=AXIS2_PLACEMENT_3D('',#16457,#13157,#13158);
#11434=AXIS2_PLACEMENT_3D('',#16459,#13159,#13160);
#11435=AXIS2_PLACEMENT_3D('',#16462,#13162,#13163);
#11436=AXIS2_PLACEMENT_3D('',#16463,#13164,#13165);
#11437=AXIS2_PLACEMENT_3D('',#16465,#13166,#13167);
#11438=AXIS2_PLACEMENT_3D('',#16468,#13169,#13170);
#11439=AXIS2_PLACEMENT_3D('',#16469,#13171,#13172);
#11440=AXIS2_PLACEMENT_3D('',#16471,#13173,#13174);
#11441=AXIS2_PLACEMENT_3D('',#16474,#13176,#13177);
#11442=AXIS2_PLACEMENT_3D('',#16475,#13178,#13179);
#11443=AXIS2_PLACEMENT_3D('',#16477,#13180,#13181);
#11444=AXIS2_PLACEMENT_3D('',#16480,#13183,#13184);
#11445=AXIS2_PLACEMENT_3D('',#16481,#13185,#13186);
#11446=AXIS2_PLACEMENT_3D('',#16483,#13187,#13188);
#11447=AXIS2_PLACEMENT_3D('',#16486,#13190,#13191);
#11448=AXIS2_PLACEMENT_3D('',#16487,#13192,#13193);
#11449=AXIS2_PLACEMENT_3D('',#16489,#13194,#13195);
#11450=AXIS2_PLACEMENT_3D('',#16492,#13197,#13198);
#11451=AXIS2_PLACEMENT_3D('',#16493,#13199,#13200);
#11452=AXIS2_PLACEMENT_3D('',#16495,#13201,#13202);
#11453=AXIS2_PLACEMENT_3D('',#16498,#13204,#13205);
#11454=AXIS2_PLACEMENT_3D('',#16499,#13206,#13207);
#11455=AXIS2_PLACEMENT_3D('',#16501,#13208,#13209);
#11456=AXIS2_PLACEMENT_3D('',#16504,#13211,#13212);
#11457=AXIS2_PLACEMENT_3D('',#16505,#13213,#13214);
#11458=AXIS2_PLACEMENT_3D('',#16514,#13219,#13220);
#11459=AXIS2_PLACEMENT_3D('',#16523,#13225,#13226);
#11460=AXIS2_PLACEMENT_3D('',#16532,#13231,#13232);
#11461=AXIS2_PLACEMENT_3D('',#16533,#13233,#13234);
#11462=AXIS2_PLACEMENT_3D('',#16534,#13235,#13236);
#11463=AXIS2_PLACEMENT_3D('',#16535,#13237,#13238);
#11464=AXIS2_PLACEMENT_3D('',#16536,#13239,#13240);
#11465=AXIS2_PLACEMENT_3D('',#16537,#13241,#13242);
#11466=AXIS2_PLACEMENT_3D('',#16538,#13243,#13244);
#11467=AXIS2_PLACEMENT_3D('',#16547,#13249,#13250);
#11468=AXIS2_PLACEMENT_3D('',#16549,#13251,#13252);
#11469=AXIS2_PLACEMENT_3D('',#16552,#13254,#13255);
#11470=AXIS2_PLACEMENT_3D('',#16553,#13256,#13257);
#11471=AXIS2_PLACEMENT_3D('',#16559,#13261,#13262);
#11472=AXIS2_PLACEMENT_3D('',#16561,#13263,#13264);
#11473=AXIS2_PLACEMENT_3D('',#16564,#13266,#13267);
#11474=AXIS2_PLACEMENT_3D('',#16565,#13268,#13269);
#11475=AXIS2_PLACEMENT_3D('',#16571,#13273,#13274);
#11476=AXIS2_PLACEMENT_3D('',#16573,#13275,#13276);
#11477=AXIS2_PLACEMENT_3D('',#16576,#13278,#13279);
#11478=AXIS2_PLACEMENT_3D('',#16577,#13280,#13281);
#11479=AXIS2_PLACEMENT_3D('',#16583,#13285,#13286);
#11480=AXIS2_PLACEMENT_3D('',#16584,#13287,#13288);
#11481=AXIS2_PLACEMENT_3D('',#16585,#13289,#13290);
#11482=AXIS2_PLACEMENT_3D('',#16586,#13291,#13292);
#11483=AXIS2_PLACEMENT_3D('',#16595,#13297,#13298);
#11484=AXIS2_PLACEMENT_3D('',#16604,#13303,#13304);
#11485=AXIS2_PLACEMENT_3D('',#16613,#13309,#13310);
#11486=AXIS2_PLACEMENT_3D('',#16622,#13315,#13316);
#11487=AXIS2_PLACEMENT_3D('',#16631,#13321,#13322);
#11488=AXIS2_PLACEMENT_3D('',#16632,#13323,#13324);
#11489=AXIS2_PLACEMENT_3D('',#16633,#13325,#13326);
#11490=AXIS2_PLACEMENT_3D('',#16634,#13327,#13328);
#11491=AXIS2_PLACEMENT_3D('',#16635,#13329,#13330);
#11492=AXIS2_PLACEMENT_3D('',#16636,#13331,#13332);
#11493=AXIS2_PLACEMENT_3D('',#16637,#13333,#13334);
#11494=AXIS2_PLACEMENT_3D('',#16638,#13335,#13336);
#11495=AXIS2_PLACEMENT_3D('',#16639,#13337,#13338);
#11496=AXIS2_PLACEMENT_3D('',#16640,#13339,#13340);
#11497=AXIS2_PLACEMENT_3D('',#16641,#13341,#13342);
#11498=AXIS2_PLACEMENT_3D('',#16642,#13343,#13344);
#11499=AXIS2_PLACEMENT_3D('',#16643,#13345,#13346);
#11500=AXIS2_PLACEMENT_3D('',#16644,#13347,#13348);
#11501=AXIS2_PLACEMENT_3D('',#16645,#13349,#13350);
#11502=AXIS2_PLACEMENT_3D('',#16646,#13351,#13352);
#11503=AXIS2_PLACEMENT_3D('',#16647,#13353,#13354);
#11504=AXIS2_PLACEMENT_3D('',#16648,#13355,#13356);
#11505=AXIS2_PLACEMENT_3D('',#16649,#13357,#13358);
#11506=AXIS2_PLACEMENT_3D('',#16650,#13359,#13360);
#11507=AXIS2_PLACEMENT_3D('',#16651,#13361,#13362);
#11508=AXIS2_PLACEMENT_3D('',#16652,#13363,#13364);
#11509=AXIS2_PLACEMENT_3D('',#16653,#13365,#13366);
#11510=AXIS2_PLACEMENT_3D('',#16654,#13367,#13368);
#13141=DIRECTION('axis',(0.,0.,1.));
#13142=DIRECTION('refdir',(1.,0.,0.));
#13143=DIRECTION('center_axis',(0.,0.,1.));
#13144=DIRECTION('ref_axis',(1.,0.,0.));
#13145=DIRECTION('center_axis',(0.,0.,1.));
#13146=DIRECTION('ref_axis',(1.,0.,0.));
#13147=DIRECTION('',(0.,0.,1.));
#13148=DIRECTION('center_axis',(0.,0.,1.));
#13149=DIRECTION('ref_axis',(1.,0.,0.));
#13150=DIRECTION('center_axis',(0.,0.,1.));
#13151=DIRECTION('ref_axis',(1.,0.,0.));
#13152=DIRECTION('center_axis',(0.,0.,1.));
#13153=DIRECTION('ref_axis',(1.,0.,0.));
#13154=DIRECTION('',(0.,0.,1.));
#13155=DIRECTION('center_axis',(0.,0.,1.));
#13156=DIRECTION('ref_axis',(1.,0.,0.));
#13157=DIRECTION('center_axis',(0.,0.,1.));
#13158=DIRECTION('ref_axis',(1.,0.,0.));
#13159=DIRECTION('center_axis',(0.,0.,1.));
#13160=DIRECTION('ref_axis',(1.,0.,0.));
#13161=DIRECTION('',(0.,0.,1.));
#13162=DIRECTION('center_axis',(0.,0.,1.));
#13163=DIRECTION('ref_axis',(1.,0.,0.));
#13164=DIRECTION('center_axis',(0.,0.,1.));
#13165=DIRECTION('ref_axis',(1.,0.,0.));
#13166=DIRECTION('center_axis',(0.,0.,1.));
#13167=DIRECTION('ref_axis',(1.,0.,0.));
#13168=DIRECTION('',(0.,0.,1.));
#13169=DIRECTION('center_axis',(0.,0.,1.));
#13170=DIRECTION('ref_axis',(1.,0.,0.));
#13171=DIRECTION('center_axis',(0.,0.,-1.));
#13172=DIRECTION('ref_axis',(-1.,0.,0.));
#13173=DIRECTION('center_axis',(0.,0.,-1.));
#13174=DIRECTION('ref_axis',(-1.,0.,0.));
#13175=DIRECTION('',(0.,0.,-1.));
#13176=DIRECTION('center_axis',(0.,0.,1.));
#13177=DIRECTION('ref_axis',(-1.,0.,0.));
#13178=DIRECTION('center_axis',(0.,0.,1.));
#13179=DIRECTION('ref_axis',(1.,0.,0.));
#13180=DIRECTION('center_axis',(0.,0.,1.));
#13181=DIRECTION('ref_axis',(-1.,0.,0.));
#13182=DIRECTION('',(0.,0.,1.));
#13183=DIRECTION('center_axis',(0.,0.,1.));
#13184=DIRECTION('ref_axis',(-1.,0.,0.));
#13185=DIRECTION('center_axis',(0.,0.,1.));
#13186=DIRECTION('ref_axis',(1.,0.,0.));
#13187=DIRECTION('center_axis',(0.,0.,1.));
#13188=DIRECTION('ref_axis',(-1.,0.,0.));
#13189=DIRECTION('',(0.,0.,1.));
#13190=DIRECTION('center_axis',(0.,0.,1.));
#13191=DIRECTION('ref_axis',(-1.,0.,0.));
#13192=DIRECTION('center_axis',(0.,0.,1.));
#13193=DIRECTION('ref_axis',(1.,0.,0.));
#13194=DIRECTION('center_axis',(0.,0.,1.));
#13195=DIRECTION('ref_axis',(-1.,0.,0.));
#13196=DIRECTION('',(0.,0.,1.));
#13197=DIRECTION('center_axis',(0.,0.,1.));
#13198=DIRECTION('ref_axis',(1.,0.,0.));
#13199=DIRECTION('center_axis',(0.,0.,1.));
#13200=DIRECTION('ref_axis',(1.,0.,0.));
#13201=DIRECTION('center_axis',(0.,0.,1.));
#13202=DIRECTION('ref_axis',(-1.,0.,0.));
#13203=DIRECTION('',(0.,0.,1.));
#13204=DIRECTION('center_axis',(0.,0.,1.));
#13205=DIRECTION('ref_axis',(1.,0.,0.));
#13206=DIRECTION('center_axis',(0.,0.,1.));
#13207=DIRECTION('ref_axis',(1.,0.,0.));
#13208=DIRECTION('center_axis',(0.,0.,1.));
#13209=DIRECTION('ref_axis',(-1.,0.,0.));
#13210=DIRECTION('',(0.,0.,1.));
#13211=DIRECTION('center_axis',(0.,0.,1.));
#13212=DIRECTION('ref_axis',(1.,0.,0.));
#13213=DIRECTION('center_axis',(-1.,2.77555756156289E-16,0.));
#13214=DIRECTION('ref_axis',(-2.77555756156289E-16,-1.,0.));
#13215=DIRECTION('',(-3.31545529486744E-16,-1.,0.));
#13216=DIRECTION('',(0.,0.,1.));
#13217=DIRECTION('',(-4.78544407166016E-16,1.,0.));
#13218=DIRECTION('',(0.,0.,-1.));
#13219=DIRECTION('center_axis',(0.,-1.,0.));
#13220=DIRECTION('ref_axis',(0.,0.,-1.));
#13221=DIRECTION('',(1.,0.,0.));
#13222=DIRECTION('',(0.,0.,1.));
#13223=DIRECTION('',(-1.,0.,0.));
#13224=DIRECTION('',(0.,0.,-1.));
#13225=DIRECTION('center_axis',(1.,0.,0.));
#13226=DIRECTION('ref_axis',(0.,0.,-1.));
#13227=DIRECTION('',(0.,1.,0.));
#13228=DIRECTION('',(0.,0.,1.));
#13229=DIRECTION('',(0.,-1.,0.));
#13230=DIRECTION('',(0.,0.,-1.));
#13231=DIRECTION('center_axis',(0.,0.,-1.));
#13232=DIRECTION('ref_axis',(-1.,0.,0.));
#13233=DIRECTION('center_axis',(0.,0.,-1.));
#13234=DIRECTION('ref_axis',(-1.,0.,0.));
#13235=DIRECTION('center_axis',(0.,0.,1.));
#13236=DIRECTION('ref_axis',(1.,0.,0.));
#13237=DIRECTION('center_axis',(0.,0.,-1.));
#13238=DIRECTION('ref_axis',(-1.,0.,0.));
#13239=DIRECTION('center_axis',(0.,0.,-1.));
#13240=DIRECTION('ref_axis',(-1.,0.,0.));
#13241=DIRECTION('center_axis',(0.,0.,1.));
#13242=DIRECTION('ref_axis',(1.,0.,0.));
#13243=DIRECTION('center_axis',(0.,-1.,0.));
#13244=DIRECTION('ref_axis',(0.,0.,-1.));
#13245=DIRECTION('',(0.,0.,1.));
#13246=DIRECTION('',(1.,0.,0.));
#13247=DIRECTION('',(0.,0.,1.));
#13248=DIRECTION('',(1.,0.,0.));
#13249=DIRECTION('center_axis',(0.,0.,1.));
#13250=DIRECTION('ref_axis',(1.,0.,0.));
#13251=DIRECTION('center_axis',(0.,0.,1.));
#13252=DIRECTION('ref_axis',(-1.,0.,0.));
#13253=DIRECTION('',(0.,0.,1.));
#13254=DIRECTION('center_axis',(0.,0.,1.));
#13255=DIRECTION('ref_axis',(1.,0.,0.));
#13256=DIRECTION('center_axis',(-1.,-1.44560289664734E-16,0.));
#13257=DIRECTION('ref_axis',(1.44560289664734E-16,-1.,0.));
#13258=DIRECTION('',(1.44560289664734E-16,-1.,0.));
#13259=DIRECTION('',(0.,0.,1.));
#13260=DIRECTION('',(1.44560289664734E-16,-1.,0.));
#13261=DIRECTION('center_axis',(0.,0.,1.));
#13262=DIRECTION('ref_axis',(1.,0.,0.));
#13263=DIRECTION('center_axis',(0.,0.,1.));
#13264=DIRECTION('ref_axis',(-1.,1.15648231731787E-15,0.));
#13265=DIRECTION('',(0.,0.,1.));
#13266=DIRECTION('center_axis',(0.,0.,1.));
#13267=DIRECTION('ref_axis',(1.,0.,0.));
#13268=DIRECTION('center_axis',(0.,-1.,0.));
#13269=DIRECTION('ref_axis',(0.,0.,-1.));
#13270=DIRECTION('',(1.,0.,0.));
#13271=DIRECTION('',(0.,0.,1.));
#13272=DIRECTION('',(1.,0.,0.));
#13273=DIRECTION('center_axis',(0.,0.,1.));
#13274=DIRECTION('ref_axis',(1.,0.,0.));
#13275=DIRECTION('center_axis',(0.,0.,1.));
#13276=DIRECTION('ref_axis',(-1.,0.,0.));
#13277=DIRECTION('',(0.,0.,1.));
#13278=DIRECTION('center_axis',(0.,0.,1.));
#13279=DIRECTION('ref_axis',(1.,0.,0.));
#13280=DIRECTION('center_axis',(-1.,-1.44560289664734E-16,0.));
#13281=DIRECTION('ref_axis',(1.44560289664734E-16,-1.,0.));
#13282=DIRECTION('',(1.44560289664734E-16,-1.,0.));
#13283=DIRECTION('',(0.,0.,1.));
#13284=DIRECTION('',(1.44560289664734E-16,-1.,0.));
#13285=DIRECTION('center_axis',(0.,0.,1.));
#13286=DIRECTION('ref_axis',(1.,0.,0.));
#13287=DIRECTION('center_axis',(0.,0.,1.));
#13288=DIRECTION('ref_axis',(-1.,0.,0.));
#13289=DIRECTION('center_axis',(0.,0.,1.));
#13290=DIRECTION('ref_axis',(1.,0.,0.));
#13291=DIRECTION('center_axis',(-1.,-1.19636101791504E-16,0.));
#13292=DIRECTION('ref_axis',(1.19636101791504E-16,-1.,0.));
#13293=DIRECTION('',(0.,0.,-1.));
#13294=DIRECTION('',(0.,1.,0.));
#13295=DIRECTION('',(0.,0.,1.));
#13296=DIRECTION('',(1.19636101791504E-16,-1.,0.));
#13297=DIRECTION('center_axis',(-0.707106781186546,0.707106781186549,0.));
#13298=DIRECTION('ref_axis',(-0.707106781186549,-0.707106781186546,0.));
#13299=DIRECTION('',(0.,0.,-1.));
#13300=DIRECTION('',(0.707106781186549,0.707106781186546,0.));
#13301=DIRECTION('',(0.,0.,1.));
#13302=DIRECTION('',(-0.707106781186549,-0.707106781186546,0.));
#13303=DIRECTION('center_axis',(0.,-1.,0.));
#13304=DIRECTION('ref_axis',(0.,0.,-1.));
#13305=DIRECTION('',(0.,0.,-1.));
#13306=DIRECTION('',(-1.,6.42490176287706E-17,0.));
#13307=DIRECTION('',(0.,0.,1.));
#13308=DIRECTION('',(1.,0.,0.));
#13309=DIRECTION('center_axis',(1.,0.,0.));
#13310=DIRECTION('ref_axis',(0.,0.,-1.));
#13311=DIRECTION('',(0.,0.,-1.));
#13312=DIRECTION('',(0.,-1.,0.));
#13313=DIRECTION('',(0.,0.,1.));
#13314=DIRECTION('',(0.,1.,0.));
#13315=DIRECTION('center_axis',(0.707106781186547,-0.707106781186548,0.));
#13316=DIRECTION('ref_axis',(0.707106781186548,0.707106781186547,0.));
#13317=DIRECTION('',(0.,0.,-1.));
#13318=DIRECTION('',(-0.707106781186549,-0.707106781186546,0.));
#13319=DIRECTION('',(0.,0.,1.));
#13320=DIRECTION('',(0.707106781186548,0.707106781186547,0.));
#13321=DIRECTION('center_axis',(0.,0.,1.));
#13322=DIRECTION('ref_axis',(1.,0.,0.));
#13323=DIRECTION('center_axis',(0.,0.,-1.));
#13324=DIRECTION('ref_axis',(-1.,0.,0.));
#13325=DIRECTION('center_axis',(0.,0.,1.));
#13326=DIRECTION('ref_axis',(1.,0.,0.));
#13327=DIRECTION('center_axis',(0.,0.,-1.));
#13328=DIRECTION('ref_axis',(-1.,0.,0.));
#13329=DIRECTION('center_axis',(0.,0.,1.));
#13330=DIRECTION('ref_axis',(-1.,0.,0.));
#13331=DIRECTION('center_axis',(0.,0.,-1.));
#13332=DIRECTION('ref_axis',(1.,1.73472347597681E-15,0.));
#13333=DIRECTION('center_axis',(0.,0.,1.));
#13334=DIRECTION('ref_axis',(1.,0.,0.));
#13335=DIRECTION('center_axis',(0.,0.,-1.));
#13336=DIRECTION('ref_axis',(-1.,0.,0.));
#13337=DIRECTION('center_axis',(0.,0.,1.));
#13338=DIRECTION('ref_axis',(1.,0.,0.));
#13339=DIRECTION('center_axis',(0.,0.,1.));
#13340=DIRECTION('ref_axis',(1.,0.,0.));
#13341=DIRECTION('center_axis',(0.,0.,-1.));
#13342=DIRECTION('ref_axis',(-1.,0.,0.));
#13343=DIRECTION('center_axis',(0.,0.,1.));
#13344=DIRECTION('ref_axis',(1.,0.,0.));
#13345=DIRECTION('center_axis',(0.,0.,1.));
#13346=DIRECTION('ref_axis',(1.,0.,0.));
#13347=DIRECTION('center_axis',(0.,0.,-1.));
#13348=DIRECTION('ref_axis',(-1.,0.,0.));
#13349=DIRECTION('center_axis',(0.,0.,1.));
#13350=DIRECTION('ref_axis',(1.,0.,0.));
#13351=DIRECTION('center_axis',(0.,0.,1.));
#13352=DIRECTION('ref_axis',(1.,0.,0.));
#13353=DIRECTION('center_axis',(0.,0.,1.));
#13354=DIRECTION('ref_axis',(-1.,0.,0.));
#13355=DIRECTION('center_axis',(0.,0.,-1.));
#13356=DIRECTION('ref_axis',(1.,-2.08166817117217E-15,0.));
#13357=DIRECTION('center_axis',(0.,0.,1.));
#13358=DIRECTION('ref_axis',(1.,0.,0.));
#13359=DIRECTION('center_axis',(0.,0.,-1.));
#13360=DIRECTION('ref_axis',(-1.,0.,0.));
#13361=DIRECTION('center_axis',(0.,0.,-1.));
#13362=DIRECTION('ref_axis',(-1.,0.,0.));
#13363=DIRECTION('center_axis',(0.,0.,-1.));
#13364=DIRECTION('ref_axis',(-1.,0.,0.));
#13365=DIRECTION('center_axis',(0.,0.,-1.));
#13366=DIRECTION('ref_axis',(-1.,0.,0.));
#13367=DIRECTION('center_axis',(0.,0.,-1.));
#13368=DIRECTION('ref_axis',(-1.,0.,0.));
#16444=CARTESIAN_POINT('',(0.,0.,0.));
#16445=CARTESIAN_POINT('Origin',(9.,9.25,5.));
#16446=CARTESIAN_POINT('',(6.,9.25,1.6));
#16447=CARTESIAN_POINT('Origin',(9.,9.25,1.6));
#16448=CARTESIAN_POINT('',(6.,9.25,5.));
#16449=CARTESIAN_POINT('',(6.,9.25,5.));
#16450=CARTESIAN_POINT('Origin',(9.,9.25,5.));
#16451=CARTESIAN_POINT('Origin',(9.,-9.25,5.));
#16452=CARTESIAN_POINT('',(6.,-9.25,1.6));
#16453=CARTESIAN_POINT('Origin',(9.,-9.25,1.6));
#16454=CARTESIAN_POINT('',(6.,-9.25,5.));
#16455=CARTESIAN_POINT('',(6.,-9.25,5.));
#16456=CARTESIAN_POINT('Origin',(9.,-9.25,5.));
#16457=CARTESIAN_POINT('Origin',(15.7,41.,5.));
#16458=CARTESIAN_POINT('',(12.45,41.,1.6));
#16459=CARTESIAN_POINT('Origin',(15.7,41.,1.6));
#16460=CARTESIAN_POINT('',(12.45,41.,5.));
#16461=CARTESIAN_POINT('',(12.45,41.,5.));
#16462=CARTESIAN_POINT('Origin',(15.7,41.,5.));
#16463=CARTESIAN_POINT('Origin',(15.7,27.,5.));
#16464=CARTESIAN_POINT('',(12.45,27.,1.6));
#16465=CARTESIAN_POINT('Origin',(15.7,27.,1.6));
#16466=CARTESIAN_POINT('',(12.45,27.,5.));
#16467=CARTESIAN_POINT('',(12.45,27.,5.));
#16468=CARTESIAN_POINT('Origin',(15.7,27.,5.));
#16469=CARTESIAN_POINT('Origin',(-0.5,0.,5.));
#16470=CARTESIAN_POINT('',(1.75,-2.75545529808155E-16,5.));
#16471=CARTESIAN_POINT('Origin',(-0.5,0.,5.));
#16472=CARTESIAN_POINT('',(1.75,-2.75545529808155E-16,0.499999999999999));
#16473=CARTESIAN_POINT('',(1.75,-2.75545529808155E-16,5.));
#16474=CARTESIAN_POINT('Origin',(-0.5,0.,0.5));
#16475=CARTESIAN_POINT('Origin',(9.,-9.25,-5.));
#16476=CARTESIAN_POINT('',(7.25,-9.25,0.499999999999999));
#16477=CARTESIAN_POINT('Origin',(9.,-9.25,0.5));
#16478=CARTESIAN_POINT('',(7.25,-9.25,1.6));
#16479=CARTESIAN_POINT('',(7.25,-9.25,-5.));
#16480=CARTESIAN_POINT('Origin',(9.,-9.25,1.6));
#16481=CARTESIAN_POINT('Origin',(9.,9.25,-5.));
#16482=CARTESIAN_POINT('',(7.25,9.25,0.499999999999999));
#16483=CARTESIAN_POINT('Origin',(9.,9.25,0.5));
#16484=CARTESIAN_POINT('',(7.25,9.25,1.6));
#16485=CARTESIAN_POINT('',(7.25,9.25,-5.));
#16486=CARTESIAN_POINT('Origin',(9.,9.25,1.6));
#16487=CARTESIAN_POINT('Origin',(-11.25,0.,0.));
#16488=CARTESIAN_POINT('',(-14.25,-3.67394039744206E-16,0.5));
#16489=CARTESIAN_POINT('Origin',(-11.25,0.,0.5));
#16490=CARTESIAN_POINT('',(-14.25,-3.67394039744206E-16,5.));
#16491=CARTESIAN_POINT('',(-14.25,-3.67394039744206E-16,0.));
#16492=CARTESIAN_POINT('Origin',(-11.25,0.,5.));
#16493=CARTESIAN_POINT('Origin',(15.7,41.,5.));
#16494=CARTESIAN_POINT('',(14.2,41.,0.499999999999999));
#16495=CARTESIAN_POINT('Origin',(15.7,41.,0.5));
#16496=CARTESIAN_POINT('',(14.2,41.,1.6));
#16497=CARTESIAN_POINT('',(14.2,41.,5.));
#16498=CARTESIAN_POINT('Origin',(15.7,41.,1.6));
#16499=CARTESIAN_POINT('Origin',(15.7,27.,5.));
#16500=CARTESIAN_POINT('',(14.2,27.,0.499999999999999));
#16501=CARTESIAN_POINT('Origin',(15.7,27.,0.5));
#16502=CARTESIAN_POINT('',(14.2,27.,1.6));
#16503=CARTESIAN_POINT('',(14.2,27.,5.));
#16504=CARTESIAN_POINT('Origin',(15.7,27.,1.6));
#16505=CARTESIAN_POINT('Origin',(20.,46.5,5.));
#16506=CARTESIAN_POINT('',(20.,42.5,0.5));
#16507=CARTESIAN_POINT('',(20.,21.5710678118655,0.5));
#16508=CARTESIAN_POINT('',(20.,42.5,0.5));
#16509=CARTESIAN_POINT('',(20.,42.5,5.));
#16510=CARTESIAN_POINT('',(20.,42.5,5.));
#16511=CARTESIAN_POINT('',(20.,21.5710678118655,5.));
#16512=CARTESIAN_POINT('',(20.,34.,5.));
#16513=CARTESIAN_POINT('',(20.,21.5710678118655,0.));
#16514=CARTESIAN_POINT('Origin',(-12.5,46.5,5.));
#16515=CARTESIAN_POINT('',(-8.5,46.5,0.5));
#16516=CARTESIAN_POINT('',(16.,46.5,0.5));
#16517=CARTESIAN_POINT('',(-8.5,46.5,0.5));
#16518=CARTESIAN_POINT('',(-8.5,46.5,5.));
#16519=CARTESIAN_POINT('',(-8.5,46.5,5.));
#16520=CARTESIAN_POINT('',(16.,46.5,5.));
#16521=CARTESIAN_POINT('',(-12.5,46.5,5.));
#16522=CARTESIAN_POINT('',(16.,46.5,5.));
#16523=CARTESIAN_POINT('Origin',(-12.5,0.,5.));
#16524=CARTESIAN_POINT('',(-12.5,28.5710678118655,0.5));
#16525=CARTESIAN_POINT('',(-12.5,42.5,0.5));
#16526=CARTESIAN_POINT('',(-12.5,28.5710678118655,0.5));
#16527=CARTESIAN_POINT('',(-12.5,28.5710678118655,5.));
#16528=CARTESIAN_POINT('',(-12.5,28.5710678118655,5.));
#16529=CARTESIAN_POINT('',(-12.5,42.5,5.));
#16530=CARTESIAN_POINT('',(-12.5,0.,5.));
#16531=CARTESIAN_POINT('',(-12.5,42.5,5.));
#16532=CARTESIAN_POINT('Origin',(-8.5,42.5,5.));
#16533=CARTESIAN_POINT('Origin',(-8.5,42.5,0.5));
#16534=CARTESIAN_POINT('Origin',(-8.5,42.5,5.));
#16535=CARTESIAN_POINT('Origin',(16.,42.5,5.));
#16536=CARTESIAN_POINT('Origin',(16.,42.5,0.5));
#16537=CARTESIAN_POINT('Origin',(16.,42.5,5.));
#16538=CARTESIAN_POINT('Origin',(0.,40.5,0.));
#16539=CARTESIAN_POINT('',(-4.,40.5,0.5));
#16540=CARTESIAN_POINT('',(-4.,40.5,5.));
#16541=CARTESIAN_POINT('',(-4.,40.5,0.));
#16542=CARTESIAN_POINT('',(4.,40.5,0.5));
#16543=CARTESIAN_POINT('',(0.,40.5,0.5));
#16544=CARTESIAN_POINT('',(4.,40.5,5.));
#16545=CARTESIAN_POINT('',(4.,40.5,0.));
#16546=CARTESIAN_POINT('',(0.,40.5,5.));
#16547=CARTESIAN_POINT('Origin',(4.,37.5,0.));
#16548=CARTESIAN_POINT('',(7.,37.5,0.5));
#16549=CARTESIAN_POINT('Origin',(4.,37.5,0.5));
#16550=CARTESIAN_POINT('',(7.,37.5,5.));
#16551=CARTESIAN_POINT('',(7.,37.5,0.));
#16552=CARTESIAN_POINT('Origin',(4.,37.5,5.));
#16553=CARTESIAN_POINT('Origin',(7.,1.01192202765314E-15,0.));
#16554=CARTESIAN_POINT('',(7.,25.5,0.5));
#16555=CARTESIAN_POINT('',(7.,1.01192202765314E-15,0.5));
#16556=CARTESIAN_POINT('',(7.,25.5,5.));
#16557=CARTESIAN_POINT('',(7.,25.5,0.));
#16558=CARTESIAN_POINT('',(7.,1.01192202765314E-15,5.));
#16559=CARTESIAN_POINT('Origin',(4.,25.5,0.));
#16560=CARTESIAN_POINT('',(4.,22.5,0.5));
#16561=CARTESIAN_POINT('Origin',(4.,25.5,0.5));
#16562=CARTESIAN_POINT('',(4.,22.5,5.));
#16563=CARTESIAN_POINT('',(4.,22.5,0.));
#16564=CARTESIAN_POINT('Origin',(4.,25.5,5.));
#16565=CARTESIAN_POINT('Origin',(0.,22.5,0.));
#16566=CARTESIAN_POINT('',(-4.,22.5,0.5));
#16567=CARTESIAN_POINT('',(0.,22.5,0.5));
#16568=CARTESIAN_POINT('',(-4.,22.5,5.));
#16569=CARTESIAN_POINT('',(-4.,22.5,0.));
#16570=CARTESIAN_POINT('',(0.,22.5,5.));
#16571=CARTESIAN_POINT('Origin',(-4.,25.5,0.));
#16572=CARTESIAN_POINT('',(-7.,25.5,0.5));
#16573=CARTESIAN_POINT('Origin',(-4.,25.5,0.5));
#16574=CARTESIAN_POINT('',(-7.,25.5,5.));
#16575=CARTESIAN_POINT('',(-7.,25.5,0.));
#16576=CARTESIAN_POINT('Origin',(-4.,25.5,5.));
#16577=CARTESIAN_POINT('Origin',(-7.,-1.01192202765314E-15,0.));
#16578=CARTESIAN_POINT('',(-7.,37.5,0.5));
#16579=CARTESIAN_POINT('',(-7.,-1.01192202765314E-15,0.5));
#16580=CARTESIAN_POINT('',(-7.,37.5,5.));
#16581=CARTESIAN_POINT('',(-7.,37.5,0.));
#16582=CARTESIAN_POINT('',(-7.,-1.01192202765314E-15,5.));
#16583=CARTESIAN_POINT('Origin',(-4.,37.5,0.));
#16584=CARTESIAN_POINT('Origin',(-4.,37.5,0.5));
#16585=CARTESIAN_POINT('Origin',(-4.,37.5,5.));
#16586=CARTESIAN_POINT('Origin',(-22.5,-2.69181229030884E-15,0.));
#16587=CARTESIAN_POINT('',(-22.5,14.4289321881346,5.));
#16588=CARTESIAN_POINT('',(-22.5,14.4289321881346,0.5));
#16589=CARTESIAN_POINT('',(-22.5,14.4289321881346,0.));
#16590=CARTESIAN_POINT('',(-22.5,-7.5,0.5));
#16591=CARTESIAN_POINT('',(-22.5,-7.5,0.5));
#16592=CARTESIAN_POINT('',(-22.5,-7.5,5.));
#16593=CARTESIAN_POINT('',(-22.5,-7.5,0.));
#16594=CARTESIAN_POINT('',(-22.5,-2.69181229030884E-15,5.));
#16595=CARTESIAN_POINT('Origin',(-19.5,19.5,0.));
#16596=CARTESIAN_POINT('',(-13.9644660940673,25.0355339059327,5.));
#16597=CARTESIAN_POINT('',(-13.9644660940673,25.0355339059327,0.5));
#16598=CARTESIAN_POINT('',(-13.9644660940673,25.0355339059327,0.));
#16599=CARTESIAN_POINT('',(-21.0355339059327,17.9644660940673,0.5));
#16600=CARTESIAN_POINT('',(-21.0355339059327,17.9644660940673,0.5));
#16601=CARTESIAN_POINT('',(-21.0355339059327,17.9644660940673,5.));
#16602=CARTESIAN_POINT('',(-21.0355339059327,17.9644660940673,0.));
#16603=CARTESIAN_POINT('',(-19.5,19.5,5.));
#16604=CARTESIAN_POINT('Origin',(0.,-12.5,0.));
#16605=CARTESIAN_POINT('',(-17.5,-12.5,5.));
#16606=CARTESIAN_POINT('',(-17.5,-12.5,0.5));
#16607=CARTESIAN_POINT('',(-17.5,-12.5,0.));
#16608=CARTESIAN_POINT('',(9.5,-12.5,0.5));
#16609=CARTESIAN_POINT('',(9.5,-12.5,0.5));
#16610=CARTESIAN_POINT('',(9.5,-12.5,5.));
#16611=CARTESIAN_POINT('',(9.5,-12.5,0.));
#16612=CARTESIAN_POINT('',(0.,-12.5,5.));
#16613=CARTESIAN_POINT('Origin',(14.5,0.,0.));
#16614=CARTESIAN_POINT('',(14.5,-7.5,5.));
#16615=CARTESIAN_POINT('',(14.5,-7.5,0.5));
#16616=CARTESIAN_POINT('',(14.5,-7.5,0.));
#16617=CARTESIAN_POINT('',(14.5,11.9289321881345,0.5));
#16618=CARTESIAN_POINT('',(14.5,11.9289321881345,0.5));
#16619=CARTESIAN_POINT('',(14.5,11.9289321881345,5.));
#16620=CARTESIAN_POINT('',(14.5,11.9289321881345,5.));
#16621=CARTESIAN_POINT('',(14.5,0.,5.));
#16622=CARTESIAN_POINT('Origin',(0.249999999999984,-0.249999999999985,0.));
#16623=CARTESIAN_POINT('',(15.9644660940673,15.4644660940673,5.));
#16624=CARTESIAN_POINT('',(15.9644660940673,15.4644660940673,0.5));
#16625=CARTESIAN_POINT('',(15.9644660940673,15.4644660940673,0.));
#16626=CARTESIAN_POINT('',(18.5355339059327,18.0355339059327,0.5));
#16627=CARTESIAN_POINT('',(18.5355339059327,18.0355339059327,0.5));
#16628=CARTESIAN_POINT('',(18.5355339059327,18.0355339059327,5.));
#16629=CARTESIAN_POINT('',(18.5355339059327,18.0355339059327,5.));
#16630=CARTESIAN_POINT('',(0.249999999999984,-0.249999999999985,5.));
#16631=CARTESIAN_POINT('Origin',(15.,21.5710678118655,5.));
#16632=CARTESIAN_POINT('Origin',(15.,21.5710678118655,0.5));
#16633=CARTESIAN_POINT('Origin',(15.,21.5710678118655,5.));
#16634=CARTESIAN_POINT('Origin',(19.5,11.9289321881345,0.));
#16635=CARTESIAN_POINT('Origin',(19.5,11.9289321881345,0.5));
#16636=CARTESIAN_POINT('Origin',(19.5,11.9289321881345,5.));
#16637=CARTESIAN_POINT('Origin',(9.5,-7.5,0.));
#16638=CARTESIAN_POINT('Origin',(9.5,-7.5,0.5));
#16639=CARTESIAN_POINT('Origin',(9.5,-7.5,5.));
#16640=CARTESIAN_POINT('Origin',(-17.5,-7.5,0.));
#16641=CARTESIAN_POINT('Origin',(-17.5,-7.5,0.5));
#16642=CARTESIAN_POINT('Origin',(-17.5,-7.5,5.));
#16643=CARTESIAN_POINT('Origin',(-17.5,14.4289321881346,0.));
#16644=CARTESIAN_POINT('Origin',(-17.5,14.4289321881346,0.5));
#16645=CARTESIAN_POINT('Origin',(-17.5,14.4289321881346,5.));
#16646=CARTESIAN_POINT('Origin',(-17.5,28.5710678118655,5.));
#16647=CARTESIAN_POINT('Origin',(-17.5,28.5710678118655,0.5));
#16648=CARTESIAN_POINT('Origin',(-17.5,28.5710678118655,5.));
#16649=CARTESIAN_POINT('Origin',(0.,1.64743813908221E-15,5.));
#16650=CARTESIAN_POINT('Origin',(17.2,27.,1.6));
#16651=CARTESIAN_POINT('Origin',(17.2,41.,1.6));
#16652=CARTESIAN_POINT('Origin',(16.,42.5,0.5));
#16653=CARTESIAN_POINT('Origin',(10.5,-9.25,1.6));
#16654=CARTESIAN_POINT('Origin',(10.5,9.25,1.6));
#18837=UNCERTAINTY_MEASURE_WITH_UNIT(LENGTH_MEASURE(0.01),#18868,
'DISTANCE_ACCURACY_VALUE',
'Maximum model space distance between geometric entities at asserted c
onnectivities');
#18849=UNCERTAINTY_MEASURE_WITH_UNIT(LENGTH_MEASURE(0.01),#18868,
'DISTANCE_ACCURACY_VALUE',
'Maximum model space distance between geometric entities at asserted c
onnectivities');
#18855=(
GEOMETRIC_REPRESENTATION_CONTEXT(3)
GLOBAL_UNCERTAINTY_ASSIGNED_CONTEXT((#18837))
GLOBAL_UNIT_ASSIGNED_CONTEXT((#18868,#18870,#18871))
REPRESENTATION_CONTEXT('','3D')
);
#18867=(
GEOMETRIC_REPRESENTATION_CONTEXT(3)
GLOBAL_UNCERTAINTY_ASSIGNED_CONTEXT((#18849))
GLOBAL_UNIT_ASSIGNED_CONTEXT((#18868,#18870,#18871))
REPRESENTATION_CONTEXT('','3D')
);
#18868=(
LENGTH_UNIT()
NAMED_UNIT(*)
SI_UNIT(.MILLI.,.METRE.)
);
#18870=(
NAMED_UNIT(*)
PLANE_ANGLE_UNIT()
SI_UNIT($,.RADIAN.)
);
#18871=(
NAMED_UNIT(*)
SI_UNIT($,.STERADIAN.)
SOLID_ANGLE_UNIT()
);
#18877=SHAPE_DEFINITION_REPRESENTATION(#18894,#18939);
#18894=PRODUCT_DEFINITION_SHAPE('',$,#18957);
#18939=SHAPE_REPRESENTATION('',(#11426),#18855);
#18951=PRODUCT_DEFINITION_CONTEXT('part definition',#19004,'design');
#18957=PRODUCT_DEFINITION('Motor Mounting Plate','Motor Mounting Plate',
#18974,#18951);
#18974=PRODUCT_DEFINITION_FORMATION('',$,#19011);
#19004=APPLICATION_CONTEXT(
'Core Data for Automotive Mechanical Design Process');
#19005=PRODUCT_CONTEXT('part definition',#19004,'mechanical');
#19011=PRODUCT('Motor Mounting Plate','Motor Mounting Plate',$,(#19005));
#19026=PRESENTATION_STYLE_ASSIGNMENT((#19032));
#19032=SURFACE_STYLE_USAGE(.BOTH.,#19038);
#19038=SURFACE_SIDE_STYLE('',(#19044));
#19044=SURFACE_STYLE_FILL_AREA(#19050);
#19050=FILL_AREA_STYLE('Opaque(227,224,212)',(#19056));
#19056=FILL_AREA_STYLE_COLOUR('Opaque(227,224,212)',#19062);
#19062=COLOUR_RGB('Opaque(227,224,212)',0.890196078431372,0.87843137254902,
0.831372549019608);
ENDSEC;
END-ISO-10303-21;
